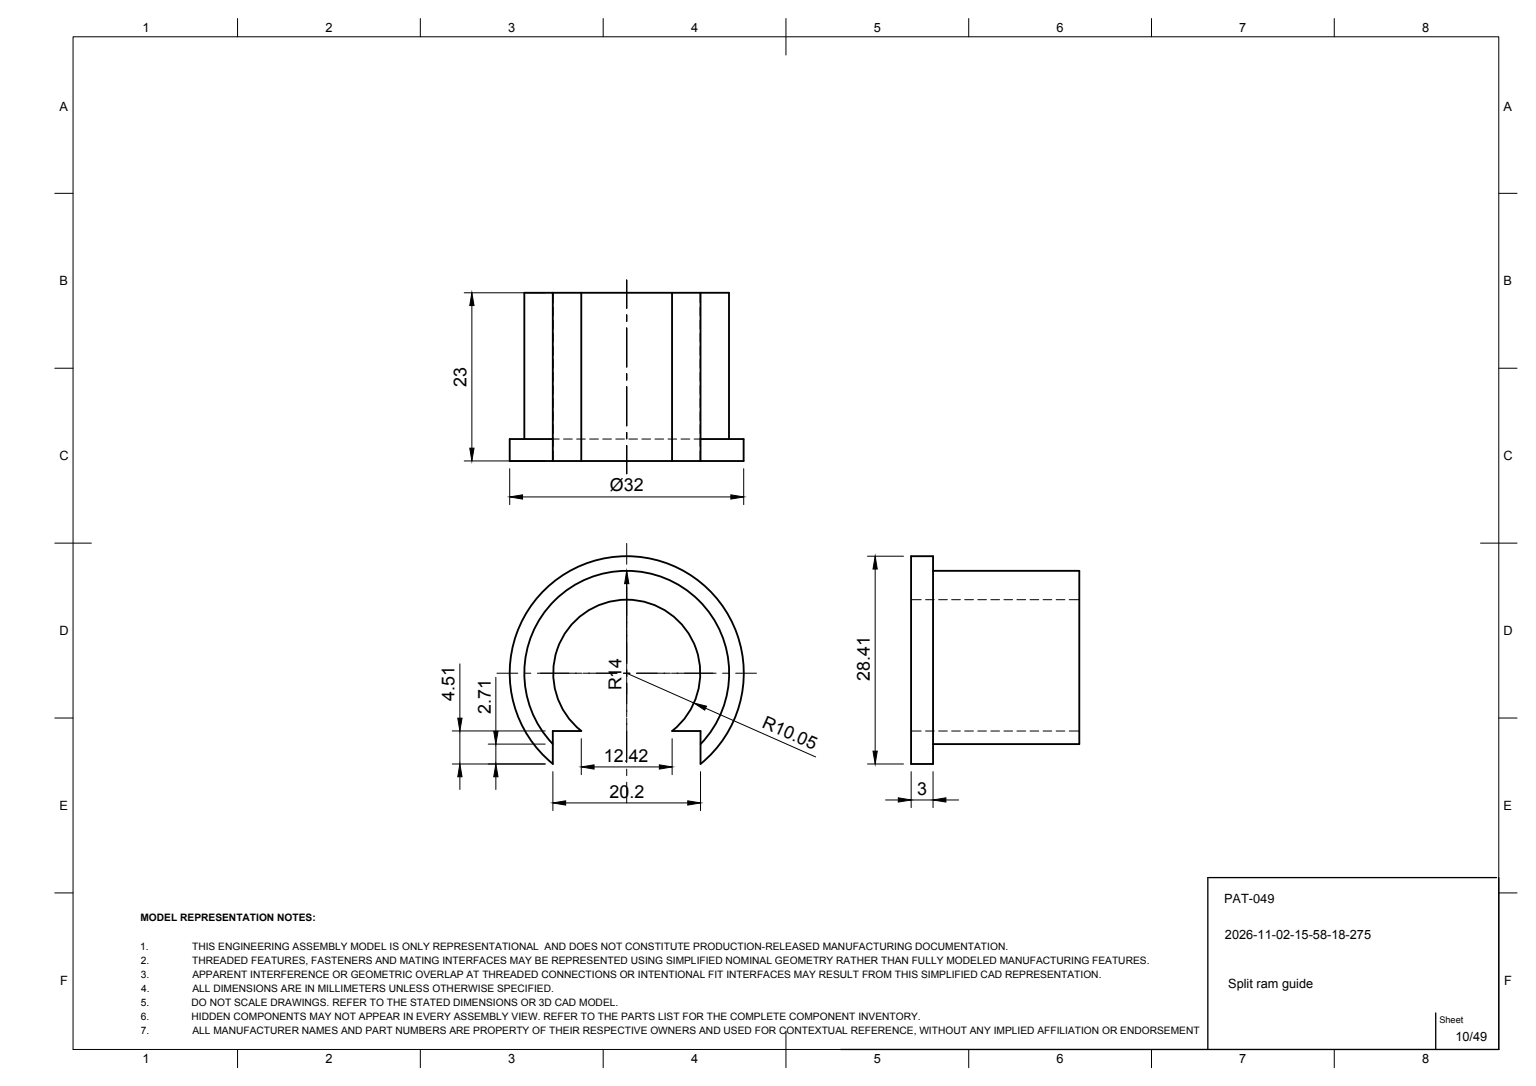
ISO-10303-21;
HEADER;
/* Generated by software containing ST-Developer
 * from STEP Tools, Inc. (www.steptools.com) 
 */

FILE_DESCRIPTION(
/* description */ ('Hand drill press frame (manual)'),
/* implementation_level */ '2;1');

FILE_NAME(
/* name */ 'Split ram guide.step',
/* time_stamp */ '2026-10-28T03:25:28-07:00',
/* author */ (''),
/* organization */ (''),
/* preprocessor_version */ 'ST-DEVELOPER v20.2',
/* originating_system */ 'Autodesk Translation Framework v15.17.0.0',
/* authorisation */ '');

FILE_SCHEMA (('AUTOMOTIVE_DESIGN { 1 0 10303 214 3 1 1 }'));
ENDSEC;

DATA;
#10=MECHANICAL_DESIGN_GEOMETRIC_PRESENTATION_REPRESENTATION('',(#624),#33299);
#534=SHAPE_REPRESENTATION_RELATIONSHIP('SRR','None',#33493,#579);
#579=ADVANCED_BREP_SHAPE_REPRESENTATION('',(#676),#33255);
#624=STYLED_ITEM('',(#33807),#676);
#676=MANIFOLD_SOLID_BREP('Body1',#12642);
#938=PLANE('',#13334);
#939=PLANE('',#13335);
#940=PLANE('',#13336);
#941=PLANE('',#13337);
#942=PLANE('',#13338);
#943=PLANE('',#13345);
#944=PLANE('',#13349);
#1417=FACE_OUTER_BOUND('',#2135,.T.);
#1418=FACE_OUTER_BOUND('',#2136,.T.);
#1419=FACE_OUTER_BOUND('',#2137,.T.);
#1420=FACE_OUTER_BOUND('',#2138,.T.);
#1421=FACE_OUTER_BOUND('',#2139,.T.);
#1422=FACE_OUTER_BOUND('',#2140,.T.);
#1423=FACE_OUTER_BOUND('',#2141,.T.);
#1424=FACE_OUTER_BOUND('',#2142,.T.);
#1425=FACE_OUTER_BOUND('',#2143,.T.);
#1426=FACE_OUTER_BOUND('',#2144,.T.);
#2135=EDGE_LOOP('',(#8787,#8788,#8789,#8790));
#2136=EDGE_LOOP('',(#8791,#8792,#8793,#8794));
#2137=EDGE_LOOP('',(#8795,#8796,#8797,#8798,#8799,#8800));
#2138=EDGE_LOOP('',(#8801,#8802,#8803,#8804,#8805,#8806));
#2139=EDGE_LOOP('',(#8807,#8808,#8809,#8810,#8811,#8812));
#2140=EDGE_LOOP('',(#8813,#8814,#8815,#8816));
#2141=EDGE_LOOP('',(#8817,#8818,#8819,#8820));
#2142=EDGE_LOOP('',(#8821,#8822,#8823,#8824));
#2143=EDGE_LOOP('',(#8825,#8826,#8827,#8828));
#2144=EDGE_LOOP('',(#8829,#8830,#8831,#8832,#8833,#8834));
#2997=LINE('',#18406,#4162);
#2998=LINE('',#18408,#4163);
#2999=LINE('',#18410,#4164);
#3000=LINE('',#18411,#4165);
#3001=LINE('',#18415,#4166);
#3002=LINE('',#18417,#4167);
#3003=LINE('',#18419,#4168);
#3004=LINE('',#18420,#4169);
#3005=LINE('',#18423,#4170);
#3006=LINE('',#18425,#4171);
#3007=LINE('',#18427,#4172);
#3008=LINE('',#18429,#4173);
#3009=LINE('',#18430,#4174);
#3010=LINE('',#18433,#4175);
#3011=LINE('',#18435,#4176);
#3012=LINE('',#18437,#4177);
#3013=LINE('',#18439,#4178);
#3014=LINE('',#18440,#4179);
#4162=VECTOR('',#14774,1.);
#4163=VECTOR('',#14775,1.);
#4164=VECTOR('',#14776,1.);
#4165=VECTOR('',#14777,1.);
#4166=VECTOR('',#14780,1.);
#4167=VECTOR('',#14781,1.);
#4168=VECTOR('',#14782,1.);
#4169=VECTOR('',#14783,1.);
#4170=VECTOR('',#14786,1.);
#4171=VECTOR('',#14787,1.);
#4172=VECTOR('',#14788,1.);
#4173=VECTOR('',#14789,1.);
#4174=VECTOR('',#14790,1.);
#4175=VECTOR('',#14793,1.);
#4176=VECTOR('',#14794,1.);
#4177=VECTOR('',#14795,1.);
#4178=VECTOR('',#14796,1.);
#4179=VECTOR('',#14797,1.);
#5274=CIRCLE('',#13339,1.4);
#5275=CIRCLE('',#13340,1.005);
#5276=CIRCLE('',#13342,1.005);
#5277=CIRCLE('',#13344,1.4);
#5278=CIRCLE('',#13346,1.6);
#5279=CIRCLE('',#13348,1.6);
#5735=VERTEX_POINT('',#18404);
#5736=VERTEX_POINT('',#18405);
#5737=VERTEX_POINT('',#18407);
#5738=VERTEX_POINT('',#18409);
#5739=VERTEX_POINT('',#18413);
#5740=VERTEX_POINT('',#18414);
#5741=VERTEX_POINT('',#18416);
#5742=VERTEX_POINT('',#18418);
#5743=VERTEX_POINT('',#18422);
#5744=VERTEX_POINT('',#18424);
#5745=VERTEX_POINT('',#18426);
#5746=VERTEX_POINT('',#18428);
#5747=VERTEX_POINT('',#18432);
#5748=VERTEX_POINT('',#18434);
#5749=VERTEX_POINT('',#18436);
#5750=VERTEX_POINT('',#18438);
#6922=EDGE_CURVE('',#5735,#5736,#2997,.T.);
#6923=EDGE_CURVE('',#5735,#5737,#2998,.T.);
#6924=EDGE_CURVE('',#5738,#5737,#2999,.T.);
#6925=EDGE_CURVE('',#5736,#5738,#3000,.T.);
#6926=EDGE_CURVE('',#5739,#5740,#3001,.T.);
#6927=EDGE_CURVE('',#5741,#5739,#3002,.T.);
#6928=EDGE_CURVE('',#5742,#5741,#3003,.T.);
#6929=EDGE_CURVE('',#5740,#5742,#3004,.T.);
#6930=EDGE_CURVE('',#5743,#5739,#3005,.T.);
#6931=EDGE_CURVE('',#5744,#5743,#3006,.T.);
#6932=EDGE_CURVE('',#5745,#5744,#3007,.T.);
#6933=EDGE_CURVE('',#5746,#5745,#3008,.T.);
#6934=EDGE_CURVE('',#5741,#5746,#3009,.T.);
#6935=EDGE_CURVE('',#5747,#5735,#3010,.T.);
#6936=EDGE_CURVE('',#5748,#5747,#3011,.T.);
#6937=EDGE_CURVE('',#5749,#5748,#3012,.T.);
#6938=EDGE_CURVE('',#5750,#5749,#3013,.T.);
#6939=EDGE_CURVE('',#5737,#5750,#3014,.T.);
#6940=EDGE_CURVE('',#5747,#5746,#5274,.T.);
#6941=EDGE_CURVE('',#5742,#5736,#5275,.T.);
#6942=EDGE_CURVE('',#5740,#5738,#5276,.T.);
#6943=EDGE_CURVE('',#5748,#5745,#5277,.T.);
#6944=EDGE_CURVE('',#5749,#5744,#5278,.T.);
#6945=EDGE_CURVE('',#5750,#5743,#5279,.T.);
#8787=ORIENTED_EDGE('',*,*,#6922,.F.);
#8788=ORIENTED_EDGE('',*,*,#6923,.T.);
#8789=ORIENTED_EDGE('',*,*,#6924,.F.);
#8790=ORIENTED_EDGE('',*,*,#6925,.F.);
#8791=ORIENTED_EDGE('',*,*,#6926,.F.);
#8792=ORIENTED_EDGE('',*,*,#6927,.F.);
#8793=ORIENTED_EDGE('',*,*,#6928,.F.);
#8794=ORIENTED_EDGE('',*,*,#6929,.F.);
#8795=ORIENTED_EDGE('',*,*,#6930,.F.);
#8796=ORIENTED_EDGE('',*,*,#6931,.F.);
#8797=ORIENTED_EDGE('',*,*,#6932,.F.);
#8798=ORIENTED_EDGE('',*,*,#6933,.F.);
#8799=ORIENTED_EDGE('',*,*,#6934,.F.);
#8800=ORIENTED_EDGE('',*,*,#6927,.T.);
#8801=ORIENTED_EDGE('',*,*,#6935,.F.);
#8802=ORIENTED_EDGE('',*,*,#6936,.F.);
#8803=ORIENTED_EDGE('',*,*,#6937,.F.);
#8804=ORIENTED_EDGE('',*,*,#6938,.F.);
#8805=ORIENTED_EDGE('',*,*,#6939,.F.);
#8806=ORIENTED_EDGE('',*,*,#6923,.F.);
#8807=ORIENTED_EDGE('',*,*,#6928,.T.);
#8808=ORIENTED_EDGE('',*,*,#6934,.T.);
#8809=ORIENTED_EDGE('',*,*,#6940,.F.);
#8810=ORIENTED_EDGE('',*,*,#6935,.T.);
#8811=ORIENTED_EDGE('',*,*,#6922,.T.);
#8812=ORIENTED_EDGE('',*,*,#6941,.F.);
#8813=ORIENTED_EDGE('',*,*,#6929,.T.);
#8814=ORIENTED_EDGE('',*,*,#6941,.T.);
#8815=ORIENTED_EDGE('',*,*,#6925,.T.);
#8816=ORIENTED_EDGE('',*,*,#6942,.F.);
#8817=ORIENTED_EDGE('',*,*,#6933,.T.);
#8818=ORIENTED_EDGE('',*,*,#6943,.F.);
#8819=ORIENTED_EDGE('',*,*,#6936,.T.);
#8820=ORIENTED_EDGE('',*,*,#6940,.T.);
#8821=ORIENTED_EDGE('',*,*,#6932,.T.);
#8822=ORIENTED_EDGE('',*,*,#6944,.F.);
#8823=ORIENTED_EDGE('',*,*,#6937,.T.);
#8824=ORIENTED_EDGE('',*,*,#6943,.T.);
#8825=ORIENTED_EDGE('',*,*,#6931,.T.);
#8826=ORIENTED_EDGE('',*,*,#6945,.F.);
#8827=ORIENTED_EDGE('',*,*,#6938,.T.);
#8828=ORIENTED_EDGE('',*,*,#6944,.T.);
#8829=ORIENTED_EDGE('',*,*,#6926,.T.);
#8830=ORIENTED_EDGE('',*,*,#6942,.T.);
#8831=ORIENTED_EDGE('',*,*,#6924,.T.);
#8832=ORIENTED_EDGE('',*,*,#6939,.T.);
#8833=ORIENTED_EDGE('',*,*,#6945,.T.);
#8834=ORIENTED_EDGE('',*,*,#6930,.T.);
#11812=CYLINDRICAL_SURFACE('',#13341,1.005);
#11813=CYLINDRICAL_SURFACE('',#13343,1.4);
#11814=CYLINDRICAL_SURFACE('',#13347,1.6);
#12026=ADVANCED_FACE('',(#1417),#938,.F.);
#12027=ADVANCED_FACE('',(#1418),#939,.F.);
#12028=ADVANCED_FACE('',(#1419),#940,.F.);
#12029=ADVANCED_FACE('',(#1420),#941,.F.);
#12030=ADVANCED_FACE('',(#1421),#942,.F.);
#12031=ADVANCED_FACE('',(#1422),#11812,.F.);
#12032=ADVANCED_FACE('',(#1423),#11813,.T.);
#12033=ADVANCED_FACE('',(#1424),#943,.F.);
#12034=ADVANCED_FACE('',(#1425),#11814,.T.);
#12035=ADVANCED_FACE('',(#1426),#944,.T.);
#12642=CLOSED_SHELL('',(#12026,#12027,#12028,#12029,#12030,#12031,#12032,
#12033,#12034,#12035));
#13333=AXIS2_PLACEMENT_3D('',#18402,#14770,#14771);
#13334=AXIS2_PLACEMENT_3D('',#18403,#14772,#14773);
#13335=AXIS2_PLACEMENT_3D('',#18412,#14778,#14779);
#13336=AXIS2_PLACEMENT_3D('',#18421,#14784,#14785);
#13337=AXIS2_PLACEMENT_3D('',#18431,#14791,#14792);
#13338=AXIS2_PLACEMENT_3D('',#18441,#14798,#14799);
#13339=AXIS2_PLACEMENT_3D('',#18442,#14800,#14801);
#13340=AXIS2_PLACEMENT_3D('',#18443,#14802,#14803);
#13341=AXIS2_PLACEMENT_3D('',#18444,#14804,#14805);
#13342=AXIS2_PLACEMENT_3D('',#18445,#14806,#14807);
#13343=AXIS2_PLACEMENT_3D('',#18446,#14808,#14809);
#13344=AXIS2_PLACEMENT_3D('',#18447,#14810,#14811);
#13345=AXIS2_PLACEMENT_3D('',#18448,#14812,#14813);
#13346=AXIS2_PLACEMENT_3D('',#18449,#14814,#14815);
#13347=AXIS2_PLACEMENT_3D('',#18450,#14816,#14817);
#13348=AXIS2_PLACEMENT_3D('',#18451,#14818,#14819);
#13349=AXIS2_PLACEMENT_3D('',#18452,#14820,#14821);
#14770=DIRECTION('axis',(0.,0.,1.));
#14771=DIRECTION('refdir',(1.,0.,0.));
#14772=DIRECTION('center_axis',(1.,0.,0.));
#14773=DIRECTION('ref_axis',(0.,1.,0.));
#14774=DIRECTION('',(0.,1.,0.));
#14775=DIRECTION('',(0.,0.,1.));
#14776=DIRECTION('',(0.,-1.,0.));
#14777=DIRECTION('',(0.,0.,1.));
#14778=DIRECTION('center_axis',(1.,0.,0.));
#14779=DIRECTION('ref_axis',(0.,1.,0.));
#14780=DIRECTION('',(0.,-1.,0.));
#14781=DIRECTION('',(0.,0.,1.));
#14782=DIRECTION('',(0.,1.,0.));
#14783=DIRECTION('',(0.,0.,-1.));
#14784=DIRECTION('center_axis',(0.,1.,0.));
#14785=DIRECTION('ref_axis',(-1.,0.,0.));
#14786=DIRECTION('',(1.,0.,0.));
#14787=DIRECTION('',(0.,0.,1.));
#14788=DIRECTION('',(-1.,0.,0.));
#14789=DIRECTION('',(0.,0.,1.));
#14790=DIRECTION('',(-1.,0.,0.));
#14791=DIRECTION('center_axis',(0.,-1.,0.));
#14792=DIRECTION('ref_axis',(1.,0.,0.));
#14793=DIRECTION('',(1.,0.,0.));
#14794=DIRECTION('',(0.,0.,-1.));
#14795=DIRECTION('',(1.,0.,0.));
#14796=DIRECTION('',(0.,0.,-1.));
#14797=DIRECTION('',(-1.,0.,0.));
#14798=DIRECTION('center_axis',(0.,0.,1.));
#14799=DIRECTION('ref_axis',(1.,0.,0.));
#14800=DIRECTION('center_axis',(0.,0.,1.));
#14801=DIRECTION('ref_axis',(1.,0.,0.));
#14802=DIRECTION('center_axis',(0.,0.,-1.));
#14803=DIRECTION('ref_axis',(1.,0.,0.));
#14804=DIRECTION('center_axis',(0.,0.,1.));
#14805=DIRECTION('ref_axis',(1.,0.,0.));
#14806=DIRECTION('center_axis',(0.,0.,-1.));
#14807=DIRECTION('ref_axis',(1.,0.,0.));
#14808=DIRECTION('center_axis',(0.,0.,1.));
#14809=DIRECTION('ref_axis',(1.,0.,0.));
#14810=DIRECTION('center_axis',(0.,0.,1.));
#14811=DIRECTION('ref_axis',(1.,0.,0.));
#14812=DIRECTION('center_axis',(0.,0.,1.));
#14813=DIRECTION('ref_axis',(1.,0.,0.));
#14814=DIRECTION('center_axis',(0.,0.,1.));
#14815=DIRECTION('ref_axis',(1.,0.,0.));
#14816=DIRECTION('center_axis',(0.,0.,1.));
#14817=DIRECTION('ref_axis',(1.,0.,0.));
#14818=DIRECTION('center_axis',(0.,0.,1.));
#14819=DIRECTION('ref_axis',(1.,0.,0.));
#14820=DIRECTION('center_axis',(0.,0.,1.));
#14821=DIRECTION('ref_axis',(1.,0.,0.));
#18402=CARTESIAN_POINT('',(0.,0.,0.));
#18403=CARTESIAN_POINT('Origin',(0.21,-1.01,12.9));
#18404=CARTESIAN_POINT('',(0.21,-1.01,13.));
#18405=CARTESIAN_POINT('',(0.21,-0.621228621362538,13.));
#18406=CARTESIAN_POINT('',(0.21,-0.505,13.));
#18407=CARTESIAN_POINT('',(0.21,-1.01,15.3));
#18408=CARTESIAN_POINT('',(0.21,-1.01,12.9));
#18409=CARTESIAN_POINT('',(0.21,-0.621228621362538,15.3));
#18410=CARTESIAN_POINT('',(0.21,-0.505,15.3));
#18411=CARTESIAN_POINT('',(0.21,-0.621228621362538,13.));
#18412=CARTESIAN_POINT('Origin',(0.21,-1.01,12.9));
#18413=CARTESIAN_POINT('',(0.21,1.01,15.3));
#18414=CARTESIAN_POINT('',(0.21,0.621228621362538,15.3));
#18415=CARTESIAN_POINT('',(0.21,-0.505,15.3));
#18416=CARTESIAN_POINT('',(0.21,1.01,13.));
#18417=CARTESIAN_POINT('',(0.21,1.01,12.9));
#18418=CARTESIAN_POINT('',(0.21,0.621228621362538,13.));
#18419=CARTESIAN_POINT('',(0.21,-0.505,13.));
#18420=CARTESIAN_POINT('',(0.21,0.621228621362538,13.));
#18421=CARTESIAN_POINT('Origin',(0.21,1.01,12.9));
#18422=CARTESIAN_POINT('',(-0.240927072796786,1.01,15.3));
#18423=CARTESIAN_POINT('',(0.605,1.01,15.3));
#18424=CARTESIAN_POINT('',(-0.240927072796786,1.01,15.));
#18425=CARTESIAN_POINT('',(-0.240927072796786,1.01,15.));
#18426=CARTESIAN_POINT('',(0.0305156009506911,1.01,15.));
#18427=CARTESIAN_POINT('',(0.605,1.01,15.));
#18428=CARTESIAN_POINT('',(0.0305156009506911,1.01,13.));
#18429=CARTESIAN_POINT('',(0.0305156009506911,1.01,13.));
#18430=CARTESIAN_POINT('',(0.605,1.01,13.));
#18431=CARTESIAN_POINT('Origin',(-0.7,-1.01,12.9));
#18432=CARTESIAN_POINT('',(0.0305156009506911,-1.01,13.));
#18433=CARTESIAN_POINT('',(0.15,-1.01,13.));
#18434=CARTESIAN_POINT('',(0.0305156009506911,-1.01,15.));
#18435=CARTESIAN_POINT('',(0.0305156009506911,-1.01,13.));
#18436=CARTESIAN_POINT('',(-0.240927072796786,-1.01,15.));
#18437=CARTESIAN_POINT('',(0.15,-1.01,15.));
#18438=CARTESIAN_POINT('',(-0.240927072796786,-1.01,15.3));
#18439=CARTESIAN_POINT('',(-0.240927072796786,-1.01,15.));
#18440=CARTESIAN_POINT('',(0.15,-1.01,15.3));
#18441=CARTESIAN_POINT('Origin',(1.,0.,13.));
#18442=CARTESIAN_POINT('Origin',(1.,0.,13.));
#18443=CARTESIAN_POINT('Origin',(1.,0.,13.));
#18444=CARTESIAN_POINT('Origin',(1.,0.,13.));
#18445=CARTESIAN_POINT('Origin',(1.,0.,15.3));
#18446=CARTESIAN_POINT('Origin',(1.,0.,13.));
#18447=CARTESIAN_POINT('Origin',(1.,0.,15.));
#18448=CARTESIAN_POINT('Origin',(1.,0.,15.));
#18449=CARTESIAN_POINT('Origin',(1.,0.,15.));
#18450=CARTESIAN_POINT('Origin',(1.,0.,15.));
#18451=CARTESIAN_POINT('Origin',(1.,0.,15.3));
#18452=CARTESIAN_POINT('Origin',(1.,0.,15.3));
#33203=UNCERTAINTY_MEASURE_WITH_UNIT(LENGTH_MEASURE(0.001),#33300,
'DISTANCE_ACCURACY_VALUE',
'Maximum model space distance between geometric entities at asserted c
onnectivities');
#33247=UNCERTAINTY_MEASURE_WITH_UNIT(LENGTH_MEASURE(0.001),#33300,
'DISTANCE_ACCURACY_VALUE',
'Maximum model space distance between geometric entities at asserted c
onnectivities');
#33255=(
GEOMETRIC_REPRESENTATION_CONTEXT(3)
GLOBAL_UNCERTAINTY_ASSIGNED_CONTEXT((#33203))
GLOBAL_UNIT_ASSIGNED_CONTEXT((#33300,#33302,#33303))
REPRESENTATION_CONTEXT('','3D')
);
#33299=(
GEOMETRIC_REPRESENTATION_CONTEXT(3)
GLOBAL_UNCERTAINTY_ASSIGNED_CONTEXT((#33247))
GLOBAL_UNIT_ASSIGNED_CONTEXT((#33300,#33302,#33303))
REPRESENTATION_CONTEXT('','3D')
);
#33300=(
LENGTH_UNIT()
NAMED_UNIT(*)
SI_UNIT(.CENTI.,.METRE.)
);
#33302=(
NAMED_UNIT(*)
PLANE_ANGLE_UNIT()
SI_UNIT($,.RADIAN.)
);
#33303=(
NAMED_UNIT(*)
SI_UNIT($,.STERADIAN.)
SOLID_ANGLE_UNIT()
);
#33311=SHAPE_DEFINITION_REPRESENTATION(#33362,#33493);
#33362=PRODUCT_DEFINITION_SHAPE('',$,#33545);
#33493=SHAPE_REPRESENTATION('',(#13333),#33255);
#33537=PRODUCT_DEFINITION_CONTEXT('part definition',#33692,'design');
#33545=PRODUCT_DEFINITION('Split ram guide','Split ram guide',#33596,#33537);
#33596=PRODUCT_DEFINITION_FORMATION('',$,#33701);
#33692=APPLICATION_CONTEXT(
'Core Data for Automotive Mechanical Design Process');
#33693=PRODUCT_CONTEXT('part definition',#33692,'mechanical');
#33701=PRODUCT('Split ram guide','Split ram guide','Split ram guide',(#33693));
#33801=COLOUR_RGB('Sky Blue',0.24,0.69,0.87);
#33802=FILL_AREA_STYLE_COLOUR('',#33801);
#33803=FILL_AREA_STYLE('',(#33802));
#33804=SURFACE_STYLE_FILL_AREA(#33803);
#33805=SURFACE_SIDE_STYLE('',(#33804));
#33806=SURFACE_STYLE_USAGE(.BOTH.,#33805);
#33807=PRESENTATION_STYLE_ASSIGNMENT((#33806));
ENDSEC;
END-ISO-10303-21;
